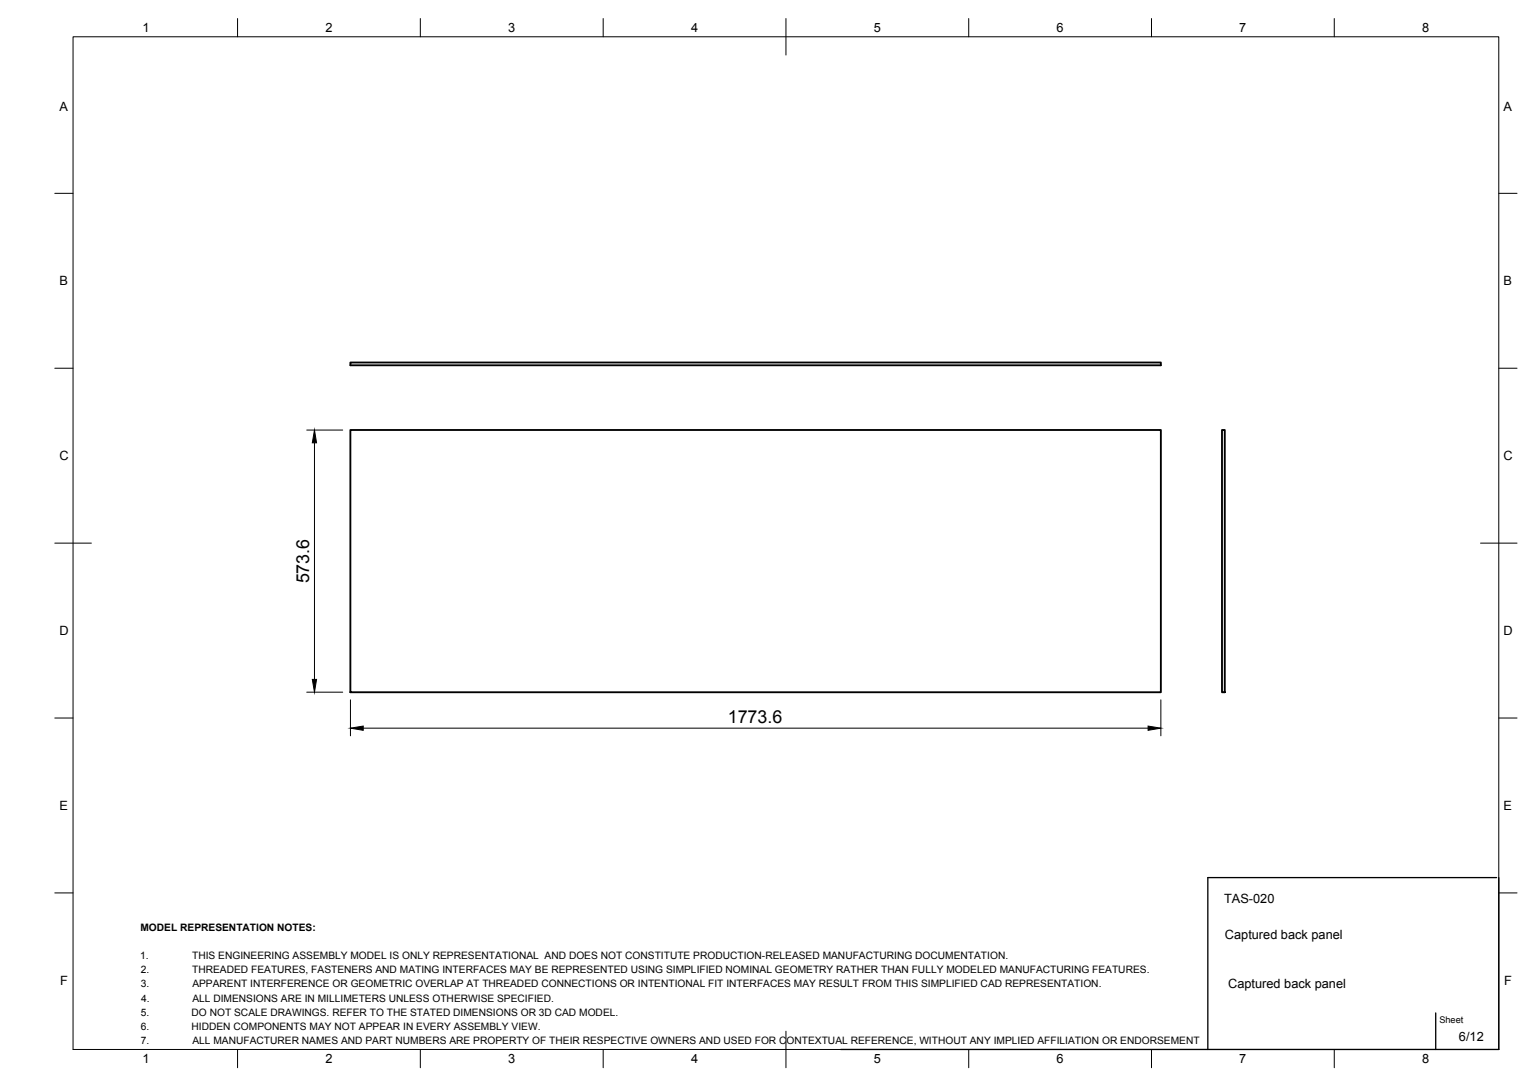
ISO-10303-21;
HEADER;
/* Generated by software containing ST-Developer
 * from STEP Tools, Inc. (www.steptools.com) 
 */

FILE_DESCRIPTION(
/* description */ (''),
/* implementation_level */ '2;1');

FILE_NAME(
/* name */ 'Captured back panel.step',
/* time_stamp */ '2026-11-15T17:46:57-08:00',
/* author */ (''),
/* organization */ (''),
/* preprocessor_version */ 'ST-DEVELOPER v20.2',
/* originating_system */ 'Autodesk Translation Framework v15.17.0.0',
/* authorisation */ '');

FILE_SCHEMA (('AUTOMOTIVE_DESIGN { 1 0 10303 214 3 1 1 }'));
ENDSEC;

DATA;
#10=MECHANICAL_DESIGN_GEOMETRIC_PRESENTATION_REPRESENTATION('',(#378),#12963);
#354=SHAPE_REPRESENTATION_RELATIONSHIP('SRR','None',#13038,#366);
#366=ADVANCED_BREP_SHAPE_REPRESENTATION('',(#390),#12954);
#378=STYLED_ITEM('',(#13107),#390);
#390=MANIFOLD_SOLID_BREP('Body1',#4812);
#505=PLANE('',#5065);
#506=PLANE('',#5066);
#507=PLANE('',#5067);
#508=PLANE('',#5068);
#509=PLANE('',#5069);
#510=PLANE('',#5070);
#650=FACE_OUTER_BOUND('',#924,.T.);
#651=FACE_OUTER_BOUND('',#925,.T.);
#652=FACE_OUTER_BOUND('',#926,.T.);
#653=FACE_OUTER_BOUND('',#927,.T.);
#654=FACE_OUTER_BOUND('',#928,.T.);
#655=FACE_OUTER_BOUND('',#929,.T.);
#924=EDGE_LOOP('',(#3484,#3485,#3486,#3487));
#925=EDGE_LOOP('',(#3488,#3489,#3490,#3491));
#926=EDGE_LOOP('',(#3492,#3493,#3494,#3495));
#927=EDGE_LOOP('',(#3496,#3497,#3498,#3499));
#928=EDGE_LOOP('',(#3500,#3501,#3502,#3503));
#929=EDGE_LOOP('',(#3504,#3505,#3506,#3507));
#1284=LINE('',#6913,#1686);
#1285=LINE('',#6915,#1687);
#1286=LINE('',#6917,#1688);
#1287=LINE('',#6918,#1689);
#1288=LINE('',#6921,#1690);
#1289=LINE('',#6923,#1691);
#1290=LINE('',#6924,#1692);
#1291=LINE('',#6927,#1693);
#1292=LINE('',#6929,#1694);
#1293=LINE('',#6930,#1695);
#1294=LINE('',#6932,#1696);
#1295=LINE('',#6933,#1697);
#1686=VECTOR('',#5723,1.);
#1687=VECTOR('',#5724,1.);
#1688=VECTOR('',#5725,1.);
#1689=VECTOR('',#5726,1.);
#1690=VECTOR('',#5729,1.);
#1691=VECTOR('',#5730,1.);
#1692=VECTOR('',#5731,1.);
#1693=VECTOR('',#5734,1.);
#1694=VECTOR('',#5735,1.);
#1695=VECTOR('',#5736,1.);
#1696=VECTOR('',#5739,1.);
#1697=VECTOR('',#5740,1.);
#2136=VERTEX_POINT('',#6911);
#2137=VERTEX_POINT('',#6912);
#2138=VERTEX_POINT('',#6914);
#2139=VERTEX_POINT('',#6916);
#2140=VERTEX_POINT('',#6920);
#2141=VERTEX_POINT('',#6922);
#2142=VERTEX_POINT('',#6926);
#2143=VERTEX_POINT('',#6928);
#2638=EDGE_CURVE('',#2136,#2137,#1284,.T.);
#2639=EDGE_CURVE('',#2137,#2138,#1285,.T.);
#2640=EDGE_CURVE('',#2139,#2138,#1286,.T.);
#2641=EDGE_CURVE('',#2136,#2139,#1287,.T.);
#2642=EDGE_CURVE('',#2140,#2136,#1288,.T.);
#2643=EDGE_CURVE('',#2141,#2139,#1289,.T.);
#2644=EDGE_CURVE('',#2140,#2141,#1290,.T.);
#2645=EDGE_CURVE('',#2142,#2140,#1291,.T.);
#2646=EDGE_CURVE('',#2143,#2141,#1292,.T.);
#2647=EDGE_CURVE('',#2142,#2143,#1293,.T.);
#2648=EDGE_CURVE('',#2137,#2142,#1294,.T.);
#2649=EDGE_CURVE('',#2138,#2143,#1295,.T.);
#3484=ORIENTED_EDGE('',*,*,#2638,.T.);
#3485=ORIENTED_EDGE('',*,*,#2639,.T.);
#3486=ORIENTED_EDGE('',*,*,#2640,.F.);
#3487=ORIENTED_EDGE('',*,*,#2641,.F.);
#3488=ORIENTED_EDGE('',*,*,#2642,.T.);
#3489=ORIENTED_EDGE('',*,*,#2641,.T.);
#3490=ORIENTED_EDGE('',*,*,#2643,.F.);
#3491=ORIENTED_EDGE('',*,*,#2644,.F.);
#3492=ORIENTED_EDGE('',*,*,#2645,.T.);
#3493=ORIENTED_EDGE('',*,*,#2644,.T.);
#3494=ORIENTED_EDGE('',*,*,#2646,.F.);
#3495=ORIENTED_EDGE('',*,*,#2647,.F.);
#3496=ORIENTED_EDGE('',*,*,#2648,.T.);
#3497=ORIENTED_EDGE('',*,*,#2647,.T.);
#3498=ORIENTED_EDGE('',*,*,#2649,.F.);
#3499=ORIENTED_EDGE('',*,*,#2639,.F.);
#3500=ORIENTED_EDGE('',*,*,#2649,.T.);
#3501=ORIENTED_EDGE('',*,*,#2646,.T.);
#3502=ORIENTED_EDGE('',*,*,#2643,.T.);
#3503=ORIENTED_EDGE('',*,*,#2640,.T.);
#3504=ORIENTED_EDGE('',*,*,#2648,.F.);
#3505=ORIENTED_EDGE('',*,*,#2638,.F.);
#3506=ORIENTED_EDGE('',*,*,#2642,.F.);
#3507=ORIENTED_EDGE('',*,*,#2645,.F.);
#4631=ADVANCED_FACE('',(#650),#505,.T.);
#4632=ADVANCED_FACE('',(#651),#506,.T.);
#4633=ADVANCED_FACE('',(#652),#507,.T.);
#4634=ADVANCED_FACE('',(#653),#508,.T.);
#4635=ADVANCED_FACE('',(#654),#509,.T.);
#4636=ADVANCED_FACE('',(#655),#510,.F.);
#4812=CLOSED_SHELL('',(#4631,#4632,#4633,#4634,#4635,#4636));
#5064=AXIS2_PLACEMENT_3D('',#6909,#5719,#5720);
#5065=AXIS2_PLACEMENT_3D('',#6910,#5721,#5722);
#5066=AXIS2_PLACEMENT_3D('',#6919,#5727,#5728);
#5067=AXIS2_PLACEMENT_3D('',#6925,#5732,#5733);
#5068=AXIS2_PLACEMENT_3D('',#6931,#5737,#5738);
#5069=AXIS2_PLACEMENT_3D('',#6934,#5741,#5742);
#5070=AXIS2_PLACEMENT_3D('',#6935,#5743,#5744);
#5719=DIRECTION('axis',(0.,0.,1.));
#5720=DIRECTION('refdir',(1.,0.,0.));
#5721=DIRECTION('center_axis',(0.,1.,0.));
#5722=DIRECTION('ref_axis',(-1.,0.,0.));
#5723=DIRECTION('',(-1.,0.,0.));
#5724=DIRECTION('',(0.,0.,1.));
#5725=DIRECTION('',(-1.,0.,0.));
#5726=DIRECTION('',(0.,0.,1.));
#5727=DIRECTION('center_axis',(1.,0.,0.));
#5728=DIRECTION('ref_axis',(0.,1.,0.));
#5729=DIRECTION('',(0.,1.,0.));
#5730=DIRECTION('',(0.,1.,0.));
#5731=DIRECTION('',(0.,0.,1.));
#5732=DIRECTION('center_axis',(0.,-1.,0.));
#5733=DIRECTION('ref_axis',(1.,0.,0.));
#5734=DIRECTION('',(1.,0.,0.));
#5735=DIRECTION('',(1.,0.,0.));
#5736=DIRECTION('',(0.,0.,1.));
#5737=DIRECTION('center_axis',(-1.,0.,0.));
#5738=DIRECTION('ref_axis',(0.,-1.,0.));
#5739=DIRECTION('',(0.,-1.,0.));
#5740=DIRECTION('',(0.,-1.,0.));
#5741=DIRECTION('center_axis',(0.,0.,1.));
#5742=DIRECTION('ref_axis',(1.,0.,0.));
#5743=DIRECTION('center_axis',(0.,0.,1.));
#5744=DIRECTION('ref_axis',(1.,0.,0.));
#6909=CARTESIAN_POINT('',(0.,0.,0.));
#6910=CARTESIAN_POINT('Origin',(57.36,0.6,0.));
#6911=CARTESIAN_POINT('',(57.36,0.6,0.));
#6912=CARTESIAN_POINT('',(0.,0.6,0.));
#6913=CARTESIAN_POINT('',(57.36,0.6,0.));
#6914=CARTESIAN_POINT('',(0.,0.6,177.36));
#6915=CARTESIAN_POINT('',(0.,0.6,0.));
#6916=CARTESIAN_POINT('',(57.36,0.6,177.36));
#6917=CARTESIAN_POINT('',(57.36,0.6,177.36));
#6918=CARTESIAN_POINT('',(57.36,0.6,0.));
#6919=CARTESIAN_POINT('Origin',(57.36,0.,0.));
#6920=CARTESIAN_POINT('',(57.36,0.,0.));
#6921=CARTESIAN_POINT('',(57.36,0.,0.));
#6922=CARTESIAN_POINT('',(57.36,0.,177.36));
#6923=CARTESIAN_POINT('',(57.36,0.,177.36));
#6924=CARTESIAN_POINT('',(57.36,0.,0.));
#6925=CARTESIAN_POINT('Origin',(0.,0.,0.));
#6926=CARTESIAN_POINT('',(0.,0.,0.));
#6927=CARTESIAN_POINT('',(0.,0.,0.));
#6928=CARTESIAN_POINT('',(0.,0.,177.36));
#6929=CARTESIAN_POINT('',(0.,0.,177.36));
#6930=CARTESIAN_POINT('',(0.,0.,0.));
#6931=CARTESIAN_POINT('Origin',(0.,0.6,0.));
#6932=CARTESIAN_POINT('',(0.,0.6,0.));
#6933=CARTESIAN_POINT('',(0.,0.6,177.36));
#6934=CARTESIAN_POINT('Origin',(28.68,0.3,177.36));
#6935=CARTESIAN_POINT('Origin',(28.68,0.3,0.));
#12940=UNCERTAINTY_MEASURE_WITH_UNIT(LENGTH_MEASURE(0.001),#12964,
'DISTANCE_ACCURACY_VALUE',
'Maximum model space distance between geometric entities at asserted c
onnectivities');
#12949=UNCERTAINTY_MEASURE_WITH_UNIT(LENGTH_MEASURE(0.001),#12964,
'DISTANCE_ACCURACY_VALUE',
'Maximum model space distance between geometric entities at asserted c
onnectivities');
#12954=(
GEOMETRIC_REPRESENTATION_CONTEXT(3)
GLOBAL_UNCERTAINTY_ASSIGNED_CONTEXT((#12940))
GLOBAL_UNIT_ASSIGNED_CONTEXT((#12964,#12966,#12967))
REPRESENTATION_CONTEXT('','3D')
);
#12963=(
GEOMETRIC_REPRESENTATION_CONTEXT(3)
GLOBAL_UNCERTAINTY_ASSIGNED_CONTEXT((#12949))
GLOBAL_UNIT_ASSIGNED_CONTEXT((#12964,#12966,#12967))
REPRESENTATION_CONTEXT('','3D')
);
#12964=(
LENGTH_UNIT()
NAMED_UNIT(*)
SI_UNIT(.CENTI.,.METRE.)
);
#12966=(
NAMED_UNIT(*)
PLANE_ANGLE_UNIT()
SI_UNIT($,.RADIAN.)
);
#12967=(
NAMED_UNIT(*)
SI_UNIT($,.STERADIAN.)
SOLID_ANGLE_UNIT()
);
#12972=SHAPE_DEFINITION_REPRESENTATION(#12985,#13038);
#12985=PRODUCT_DEFINITION_SHAPE('',$,#13052);
#13038=SHAPE_REPRESENTATION('',(#5064),#12954);
#13047=PRODUCT_DEFINITION_CONTEXT('part definition',#13088,'design');
#13052=PRODUCT_DEFINITION('Captured back panel','Captured back panel',#13065,
#13047);
#13065=PRODUCT_DEFINITION_FORMATION('',$,#13094);
#13088=APPLICATION_CONTEXT(
'Core Data for Automotive Mechanical Design Process');
#13089=PRODUCT_CONTEXT('part definition',#13088,'mechanical');
#13094=PRODUCT('Captured back panel','Captured back panel',$,(#13089));
#13107=PRESENTATION_STYLE_ASSIGNMENT((#13120));
#13120=SURFACE_STYLE_USAGE(.BOTH.,#13133);
#13133=SURFACE_SIDE_STYLE('',(#13146));
#13146=SURFACE_STYLE_FILL_AREA(#13159);
#13159=FILL_AREA_STYLE('Captured back panel finish',(#13172));
#13172=FILL_AREA_STYLE_COLOUR('Captured back panel finish',#13185);
#13185=COLOUR_RGB('Captured back panel finish',0.607843137254902,0.647058823529412,
0.701960784313725);
ENDSEC;
END-ISO-10303-21;
